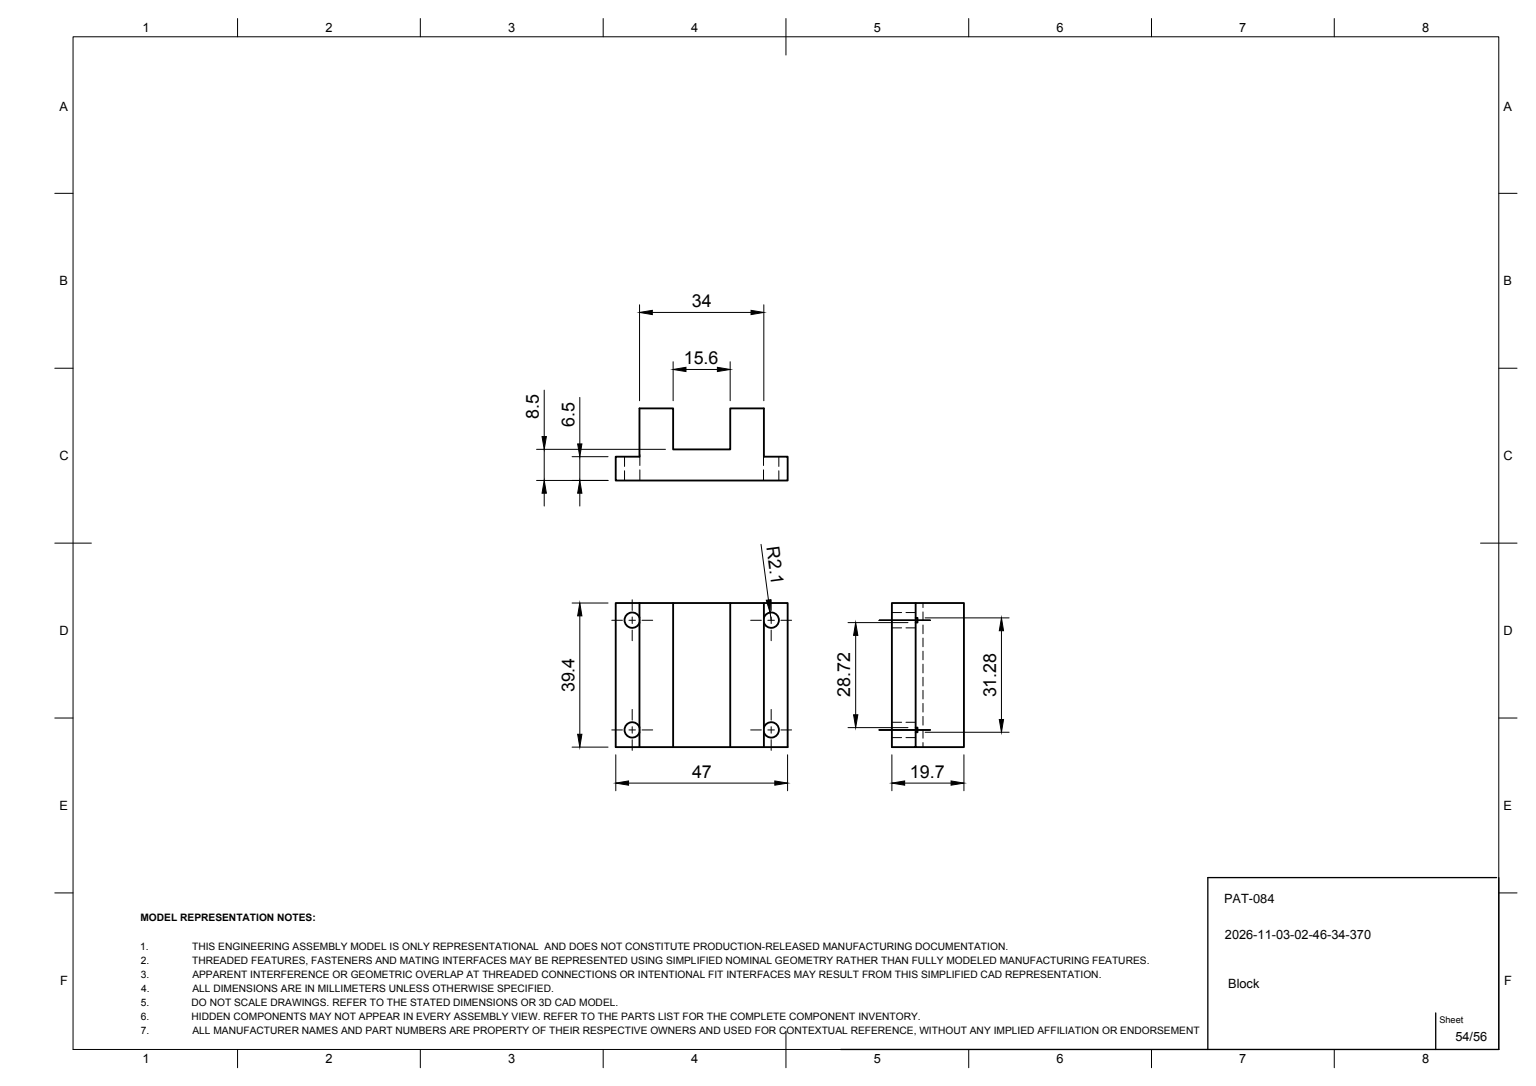
ISO-10303-21;
HEADER;
/* Generated by software containing ST-Developer
 * from STEP Tools, Inc. (www.steptools.com) 
 */

FILE_DESCRIPTION(
/* description */ ('Quick-return (Whitworth) mechanism'),
/* implementation_level */ '2;1');

FILE_NAME(
/* name */ 'Block.step',
/* time_stamp */ '2026-10-28T03:25:57-07:00',
/* author */ (''),
/* organization */ (''),
/* preprocessor_version */ 'ST-DEVELOPER v20.2',
/* originating_system */ 'Autodesk Translation Framework v15.17.0.0',
/* authorisation */ '');

FILE_SCHEMA (('AUTOMOTIVE_DESIGN { 1 0 10303 214 3 1 1 }'));
ENDSEC;

DATA;
#10=MECHANICAL_DESIGN_GEOMETRIC_PRESENTATION_REPRESENTATION('',(#537),#14878);
#441=SHAPE_REPRESENTATION_RELATIONSHIP('SRR','None',#15116,#485);
#485=ADVANCED_BREP_SHAPE_REPRESENTATION('',(#588),#14873);
#537=STYLED_ITEM('',(#15385),#588);
#588=MANIFOLD_SOLID_BREP('Body1',#7892);
#776=FACE_BOUND('',#2104,.T.);
#777=FACE_BOUND('',#2105,.T.);
#778=FACE_BOUND('',#2106,.T.);
#779=FACE_BOUND('',#2107,.T.);
#987=PLANE('',#9219);
#988=PLANE('',#9225);
#989=PLANE('',#9231);
#990=PLANE('',#9237);
#991=PLANE('',#9243);
#992=PLANE('',#9244);
#993=PLANE('',#9245);
#994=PLANE('',#9246);
#995=PLANE('',#9247);
#996=PLANE('',#9248);
#997=PLANE('',#9249);
#998=PLANE('',#9250);
#999=PLANE('',#9251);
#1000=PLANE('',#9252);
#1001=PLANE('',#9253);
#1002=PLANE('',#9254);
#1003=PLANE('',#9255);
#1004=PLANE('',#9256);
#1439=FACE_OUTER_BOUND('',#2090,.T.);
#1440=FACE_OUTER_BOUND('',#2091,.T.);
#1441=FACE_OUTER_BOUND('',#2092,.T.);
#1442=FACE_OUTER_BOUND('',#2093,.T.);
#1443=FACE_OUTER_BOUND('',#2094,.T.);
#1444=FACE_OUTER_BOUND('',#2095,.T.);
#1445=FACE_OUTER_BOUND('',#2096,.T.);
#1446=FACE_OUTER_BOUND('',#2097,.T.);
#1447=FACE_OUTER_BOUND('',#2098,.T.);
#1448=FACE_OUTER_BOUND('',#2099,.T.);
#1449=FACE_OUTER_BOUND('',#2100,.T.);
#1450=FACE_OUTER_BOUND('',#2101,.T.);
#1451=FACE_OUTER_BOUND('',#2102,.T.);
#1452=FACE_OUTER_BOUND('',#2103,.T.);
#1453=FACE_OUTER_BOUND('',#2108,.T.);
#1454=FACE_OUTER_BOUND('',#2109,.T.);
#1455=FACE_OUTER_BOUND('',#2110,.T.);
#1456=FACE_OUTER_BOUND('',#2111,.T.);
#1457=FACE_OUTER_BOUND('',#2112,.T.);
#1458=FACE_OUTER_BOUND('',#2113,.T.);
#1459=FACE_OUTER_BOUND('',#2114,.T.);
#1460=FACE_OUTER_BOUND('',#2115,.T.);
#2090=EDGE_LOOP('',(#6850,#6851));
#2091=EDGE_LOOP('',(#6852,#6853,#6854,#6855,#6856,#6857,#6858,#6859));
#2092=EDGE_LOOP('',(#6860,#6861));
#2093=EDGE_LOOP('',(#6862,#6863,#6864,#6865,#6866,#6867,#6868,#6869));
#2094=EDGE_LOOP('',(#6870,#6871));
#2095=EDGE_LOOP('',(#6872,#6873,#6874,#6875,#6876,#6877,#6878,#6879));
#2096=EDGE_LOOP('',(#6880,#6881));
#2097=EDGE_LOOP('',(#6882,#6883,#6884,#6885,#6886,#6887,#6888,#6889));
#2098=EDGE_LOOP('',(#6890,#6891,#6892,#6893,#6894,#6895,#6896,#6897,#6898,
#6899,#6900,#6901));
#2099=EDGE_LOOP('',(#6902,#6903,#6904,#6905,#6906,#6907,#6908,#6909,#6910,
#6911,#6912,#6913));
#2100=EDGE_LOOP('',(#6914,#6915,#6916,#6917,#6918,#6919,#6920,#6921,#6922,
#6923,#6924,#6925));
#2101=EDGE_LOOP('',(#6926,#6927,#6928,#6929,#6930,#6931,#6932,#6933,#6934,
#6935));
#2102=EDGE_LOOP('',(#6936,#6937,#6938,#6939));
#2103=EDGE_LOOP('',(#6940,#6941,#6942,#6943));
#2104=EDGE_LOOP('',(#6944));
#2105=EDGE_LOOP('',(#6945));
#2106=EDGE_LOOP('',(#6946));
#2107=EDGE_LOOP('',(#6947));
#2108=EDGE_LOOP('',(#6948,#6949,#6950,#6951));
#2109=EDGE_LOOP('',(#6952,#6953,#6954,#6955,#6956,#6957,#6958,#6959,#6960,
#6961));
#2110=EDGE_LOOP('',(#6962,#6963,#6964,#6965));
#2111=EDGE_LOOP('',(#6966,#6967,#6968,#6969));
#2112=EDGE_LOOP('',(#6970,#6971,#6972,#6973));
#2113=EDGE_LOOP('',(#6974,#6975,#6976,#6977));
#2114=EDGE_LOOP('',(#6978,#6979,#6980,#6981));
#2115=EDGE_LOOP('',(#6982,#6983,#6984,#6985,#6986,#6987,#6988,#6989,#6990,
#6991,#6992,#6993));
#2543=LINE('',#14328,#3066);
#2544=LINE('',#14332,#3067);
#2545=LINE('',#14336,#3068);
#2546=LINE('',#14340,#3069);
#2547=LINE('',#14344,#3070);
#2548=LINE('',#14348,#3071);
#2549=LINE('',#14352,#3072);
#2550=LINE('',#14356,#3073);
#2551=LINE('',#14360,#3074);
#2552=LINE('',#14364,#3075);
#2553=LINE('',#14368,#3076);
#2554=LINE('',#14372,#3077);
#2555=LINE('',#14376,#3078);
#2556=LINE('',#14380,#3079);
#2557=LINE('',#14384,#3080);
#2558=LINE('',#14388,#3081);
#2559=LINE('',#14390,#3082);
#2560=LINE('',#14392,#3083);
#2561=LINE('',#14394,#3084);
#2562=LINE('',#14396,#3085);
#2563=LINE('',#14398,#3086);
#2564=LINE('',#14399,#3087);
#2565=LINE('',#14401,#3088);
#2566=LINE('',#14403,#3089);
#2567=LINE('',#14405,#3090);
#2568=LINE('',#14407,#3091);
#2569=LINE('',#14409,#3092);
#2570=LINE('',#14410,#3093);
#2571=LINE('',#14413,#3094);
#2572=LINE('',#14415,#3095);
#2573=LINE('',#14417,#3096);
#2574=LINE('',#14419,#3097);
#2575=LINE('',#14420,#3098);
#2576=LINE('',#14422,#3099);
#2577=LINE('',#14424,#3100);
#2578=LINE('',#14426,#3101);
#2579=LINE('',#14428,#3102);
#2580=LINE('',#14429,#3103);
#2581=LINE('',#14432,#3104);
#2582=LINE('',#14433,#3105);
#2583=LINE('',#14436,#3106);
#2584=LINE('',#14437,#3107);
#2585=LINE('',#14440,#3108);
#2586=LINE('',#14441,#3109);
#2587=LINE('',#14444,#3110);
#2588=LINE('',#14445,#3111);
#2589=LINE('',#14447,#3112);
#2590=LINE('',#14450,#3113);
#2591=LINE('',#14451,#3114);
#2592=LINE('',#14454,#3115);
#2593=LINE('',#14455,#3116);
#2594=LINE('',#14458,#3117);
#2595=LINE('',#14459,#3118);
#2596=LINE('',#14462,#3119);
#2597=LINE('',#14463,#3120);
#2598=LINE('',#14465,#3121);
#3066=VECTOR('',#11442,1.);
#3067=VECTOR('',#11447,1.);
#3068=VECTOR('',#11450,0.21);
#3069=VECTOR('',#11455,1.);
#3070=VECTOR('',#11458,1.);
#3071=VECTOR('',#11463,1.);
#3072=VECTOR('',#11466,0.21);
#3073=VECTOR('',#11471,1.);
#3074=VECTOR('',#11474,1.);
#3075=VECTOR('',#11479,1.);
#3076=VECTOR('',#11482,0.21);
#3077=VECTOR('',#11487,1.);
#3078=VECTOR('',#11490,1.);
#3079=VECTOR('',#11495,1.);
#3080=VECTOR('',#11498,0.21);
#3081=VECTOR('',#11503,1.);
#3082=VECTOR('',#11506,1.);
#3083=VECTOR('',#11507,1.);
#3084=VECTOR('',#11508,1.);
#3085=VECTOR('',#11509,1.);
#3086=VECTOR('',#11510,1.);
#3087=VECTOR('',#11511,1.);
#3088=VECTOR('',#11514,1.);
#3089=VECTOR('',#11515,1.);
#3090=VECTOR('',#11516,1.);
#3091=VECTOR('',#11517,1.);
#3092=VECTOR('',#11518,1.);
#3093=VECTOR('',#11519,1.);
#3094=VECTOR('',#11522,1.);
#3095=VECTOR('',#11523,1.);
#3096=VECTOR('',#11524,1.);
#3097=VECTOR('',#11525,1.);
#3098=VECTOR('',#11526,1.);
#3099=VECTOR('',#11527,1.);
#3100=VECTOR('',#11528,1.);
#3101=VECTOR('',#11529,1.);
#3102=VECTOR('',#11530,1.);
#3103=VECTOR('',#11531,1.);
#3104=VECTOR('',#11534,1.);
#3105=VECTOR('',#11535,1.);
#3106=VECTOR('',#11538,1.);
#3107=VECTOR('',#11539,1.);
#3108=VECTOR('',#11542,1.);
#3109=VECTOR('',#11543,1.);
#3110=VECTOR('',#11546,1.);
#3111=VECTOR('',#11547,1.);
#3112=VECTOR('',#11550,1.);
#3113=VECTOR('',#11553,1.);
#3114=VECTOR('',#11554,1.);
#3115=VECTOR('',#11557,1.);
#3116=VECTOR('',#11558,1.);
#3117=VECTOR('',#11561,1.);
#3118=VECTOR('',#11562,1.);
#3119=VECTOR('',#11565,1.);
#3120=VECTOR('',#11566,1.);
#3121=VECTOR('',#11569,1.);
#3601=CIRCLE('',#9220,0.21);
#3602=CIRCLE('',#9222,0.21);
#3603=CIRCLE('',#9223,0.21);
#3604=CIRCLE('',#9224,0.21);
#3605=CIRCLE('',#9226,0.21);
#3606=CIRCLE('',#9228,0.21);
#3607=CIRCLE('',#9229,0.21);
#3608=CIRCLE('',#9230,0.21);
#3609=CIRCLE('',#9232,0.21);
#3610=CIRCLE('',#9234,0.21);
#3611=CIRCLE('',#9235,0.21);
#3612=CIRCLE('',#9236,0.21);
#3613=CIRCLE('',#9238,0.21);
#3614=CIRCLE('',#9240,0.21);
#3615=CIRCLE('',#9241,0.21);
#3616=CIRCLE('',#9242,0.21);
#4170=VERTEX_POINT('',#14326);
#4171=VERTEX_POINT('',#14327);
#4172=VERTEX_POINT('',#14331);
#4173=VERTEX_POINT('',#14333);
#4174=VERTEX_POINT('',#14335);
#4175=VERTEX_POINT('',#14338);
#4176=VERTEX_POINT('',#14342);
#4177=VERTEX_POINT('',#14343);
#4178=VERTEX_POINT('',#14347);
#4179=VERTEX_POINT('',#14349);
#4180=VERTEX_POINT('',#14351);
#4181=VERTEX_POINT('',#14354);
#4182=VERTEX_POINT('',#14358);
#4183=VERTEX_POINT('',#14359);
#4184=VERTEX_POINT('',#14363);
#4185=VERTEX_POINT('',#14365);
#4186=VERTEX_POINT('',#14367);
#4187=VERTEX_POINT('',#14370);
#4188=VERTEX_POINT('',#14374);
#4189=VERTEX_POINT('',#14375);
#4190=VERTEX_POINT('',#14379);
#4191=VERTEX_POINT('',#14381);
#4192=VERTEX_POINT('',#14383);
#4193=VERTEX_POINT('',#14386);
#4194=VERTEX_POINT('',#14391);
#4195=VERTEX_POINT('',#14393);
#4196=VERTEX_POINT('',#14395);
#4197=VERTEX_POINT('',#14397);
#4198=VERTEX_POINT('',#14402);
#4199=VERTEX_POINT('',#14404);
#4200=VERTEX_POINT('',#14406);
#4201=VERTEX_POINT('',#14408);
#4202=VERTEX_POINT('',#14412);
#4203=VERTEX_POINT('',#14414);
#4204=VERTEX_POINT('',#14416);
#4205=VERTEX_POINT('',#14418);
#4206=VERTEX_POINT('',#14421);
#4207=VERTEX_POINT('',#14423);
#4208=VERTEX_POINT('',#14425);
#4209=VERTEX_POINT('',#14427);
#4210=VERTEX_POINT('',#14431);
#4211=VERTEX_POINT('',#14435);
#4212=VERTEX_POINT('',#14439);
#4213=VERTEX_POINT('',#14443);
#4214=VERTEX_POINT('',#14449);
#4215=VERTEX_POINT('',#14453);
#4216=VERTEX_POINT('',#14457);
#4217=VERTEX_POINT('',#14461);
#5082=EDGE_CURVE('',#4170,#4171,#2543,.T.);
#5083=EDGE_CURVE('',#4170,#4171,#3601,.T.);
#5084=EDGE_CURVE('',#4172,#4170,#2544,.T.);
#5085=EDGE_CURVE('',#4173,#4172,#3602,.T.);
#5086=EDGE_CURVE('',#4173,#4174,#2545,.T.);
#5087=EDGE_CURVE('',#4174,#4174,#3603,.T.);
#5088=EDGE_CURVE('',#4175,#4173,#3604,.T.);
#5089=EDGE_CURVE('',#4171,#4175,#2546,.T.);
#5090=EDGE_CURVE('',#4176,#4177,#2547,.T.);
#5091=EDGE_CURVE('',#4176,#4177,#3605,.T.);
#5092=EDGE_CURVE('',#4178,#4176,#2548,.T.);
#5093=EDGE_CURVE('',#4179,#4178,#3606,.T.);
#5094=EDGE_CURVE('',#4179,#4180,#2549,.T.);
#5095=EDGE_CURVE('',#4180,#4180,#3607,.T.);
#5096=EDGE_CURVE('',#4181,#4179,#3608,.T.);
#5097=EDGE_CURVE('',#4177,#4181,#2550,.T.);
#5098=EDGE_CURVE('',#4182,#4183,#2551,.T.);
#5099=EDGE_CURVE('',#4182,#4183,#3609,.T.);
#5100=EDGE_CURVE('',#4184,#4182,#2552,.T.);
#5101=EDGE_CURVE('',#4185,#4184,#3610,.T.);
#5102=EDGE_CURVE('',#4185,#4186,#2553,.T.);
#5103=EDGE_CURVE('',#4186,#4186,#3611,.T.);
#5104=EDGE_CURVE('',#4187,#4185,#3612,.T.);
#5105=EDGE_CURVE('',#4183,#4187,#2554,.T.);
#5106=EDGE_CURVE('',#4188,#4189,#2555,.T.);
#5107=EDGE_CURVE('',#4188,#4189,#3613,.T.);
#5108=EDGE_CURVE('',#4190,#4188,#2556,.T.);
#5109=EDGE_CURVE('',#4191,#4190,#3614,.T.);
#5110=EDGE_CURVE('',#4191,#4192,#2557,.T.);
#5111=EDGE_CURVE('',#4192,#4192,#3615,.T.);
#5112=EDGE_CURVE('',#4193,#4191,#3616,.T.);
#5113=EDGE_CURVE('',#4189,#4193,#2558,.T.);
#5114=EDGE_CURVE('',#4175,#4184,#2559,.T.);
#5115=EDGE_CURVE('',#4187,#4194,#2560,.T.);
#5116=EDGE_CURVE('',#4195,#4194,#2561,.T.);
#5117=EDGE_CURVE('',#4195,#4196,#2562,.T.);
#5118=EDGE_CURVE('',#4197,#4196,#2563,.T.);
#5119=EDGE_CURVE('',#4197,#4172,#2564,.T.);
#5120=EDGE_CURVE('',#4181,#4190,#2565,.T.);
#5121=EDGE_CURVE('',#4193,#4198,#2566,.T.);
#5122=EDGE_CURVE('',#4199,#4198,#2567,.T.);
#5123=EDGE_CURVE('',#4200,#4199,#2568,.T.);
#5124=EDGE_CURVE('',#4201,#4200,#2569,.T.);
#5125=EDGE_CURVE('',#4201,#4178,#2570,.T.);
#5126=EDGE_CURVE('',#4194,#4202,#2571,.T.);
#5127=EDGE_CURVE('',#4202,#4203,#2572,.T.);
#5128=EDGE_CURVE('',#4203,#4204,#2573,.T.);
#5129=EDGE_CURVE('',#4204,#4205,#2574,.T.);
#5130=EDGE_CURVE('',#4205,#4201,#2575,.T.);
#5131=EDGE_CURVE('',#4200,#4206,#2576,.T.);
#5132=EDGE_CURVE('',#4206,#4207,#2577,.T.);
#5133=EDGE_CURVE('',#4207,#4208,#2578,.T.);
#5134=EDGE_CURVE('',#4208,#4209,#2579,.T.);
#5135=EDGE_CURVE('',#4209,#4195,#2580,.T.);
#5136=EDGE_CURVE('',#4210,#4197,#2581,.T.);
#5137=EDGE_CURVE('',#4202,#4210,#2582,.T.);
#5138=EDGE_CURVE('',#4211,#4210,#2583,.T.);
#5139=EDGE_CURVE('',#4203,#4211,#2584,.T.);
#5140=EDGE_CURVE('',#4212,#4211,#2585,.T.);
#5141=EDGE_CURVE('',#4204,#4212,#2586,.T.);
#5142=EDGE_CURVE('',#4213,#4212,#2587,.T.);
#5143=EDGE_CURVE('',#4205,#4213,#2588,.T.);
#5144=EDGE_CURVE('',#4198,#4213,#2589,.T.);
#5145=EDGE_CURVE('',#4214,#4199,#2590,.T.);
#5146=EDGE_CURVE('',#4206,#4214,#2591,.T.);
#5147=EDGE_CURVE('',#4215,#4214,#2592,.T.);
#5148=EDGE_CURVE('',#4207,#4215,#2593,.T.);
#5149=EDGE_CURVE('',#4216,#4215,#2594,.T.);
#5150=EDGE_CURVE('',#4208,#4216,#2595,.T.);
#5151=EDGE_CURVE('',#4217,#4216,#2596,.T.);
#5152=EDGE_CURVE('',#4209,#4217,#2597,.T.);
#5153=EDGE_CURVE('',#4196,#4217,#2598,.T.);
#6850=ORIENTED_EDGE('',*,*,#5082,.F.);
#6851=ORIENTED_EDGE('',*,*,#5083,.T.);
#6852=ORIENTED_EDGE('',*,*,#5084,.F.);
#6853=ORIENTED_EDGE('',*,*,#5085,.F.);
#6854=ORIENTED_EDGE('',*,*,#5086,.T.);
#6855=ORIENTED_EDGE('',*,*,#5087,.F.);
#6856=ORIENTED_EDGE('',*,*,#5086,.F.);
#6857=ORIENTED_EDGE('',*,*,#5088,.F.);
#6858=ORIENTED_EDGE('',*,*,#5089,.F.);
#6859=ORIENTED_EDGE('',*,*,#5083,.F.);
#6860=ORIENTED_EDGE('',*,*,#5090,.F.);
#6861=ORIENTED_EDGE('',*,*,#5091,.T.);
#6862=ORIENTED_EDGE('',*,*,#5092,.F.);
#6863=ORIENTED_EDGE('',*,*,#5093,.F.);
#6864=ORIENTED_EDGE('',*,*,#5094,.T.);
#6865=ORIENTED_EDGE('',*,*,#5095,.F.);
#6866=ORIENTED_EDGE('',*,*,#5094,.F.);
#6867=ORIENTED_EDGE('',*,*,#5096,.F.);
#6868=ORIENTED_EDGE('',*,*,#5097,.F.);
#6869=ORIENTED_EDGE('',*,*,#5091,.F.);
#6870=ORIENTED_EDGE('',*,*,#5098,.F.);
#6871=ORIENTED_EDGE('',*,*,#5099,.T.);
#6872=ORIENTED_EDGE('',*,*,#5100,.F.);
#6873=ORIENTED_EDGE('',*,*,#5101,.F.);
#6874=ORIENTED_EDGE('',*,*,#5102,.T.);
#6875=ORIENTED_EDGE('',*,*,#5103,.F.);
#6876=ORIENTED_EDGE('',*,*,#5102,.F.);
#6877=ORIENTED_EDGE('',*,*,#5104,.F.);
#6878=ORIENTED_EDGE('',*,*,#5105,.F.);
#6879=ORIENTED_EDGE('',*,*,#5099,.F.);
#6880=ORIENTED_EDGE('',*,*,#5106,.F.);
#6881=ORIENTED_EDGE('',*,*,#5107,.T.);
#6882=ORIENTED_EDGE('',*,*,#5108,.F.);
#6883=ORIENTED_EDGE('',*,*,#5109,.F.);
#6884=ORIENTED_EDGE('',*,*,#5110,.T.);
#6885=ORIENTED_EDGE('',*,*,#5111,.F.);
#6886=ORIENTED_EDGE('',*,*,#5110,.F.);
#6887=ORIENTED_EDGE('',*,*,#5112,.F.);
#6888=ORIENTED_EDGE('',*,*,#5113,.F.);
#6889=ORIENTED_EDGE('',*,*,#5107,.F.);
#6890=ORIENTED_EDGE('',*,*,#5084,.T.);
#6891=ORIENTED_EDGE('',*,*,#5082,.T.);
#6892=ORIENTED_EDGE('',*,*,#5089,.T.);
#6893=ORIENTED_EDGE('',*,*,#5114,.T.);
#6894=ORIENTED_EDGE('',*,*,#5100,.T.);
#6895=ORIENTED_EDGE('',*,*,#5098,.T.);
#6896=ORIENTED_EDGE('',*,*,#5105,.T.);
#6897=ORIENTED_EDGE('',*,*,#5115,.T.);
#6898=ORIENTED_EDGE('',*,*,#5116,.F.);
#6899=ORIENTED_EDGE('',*,*,#5117,.T.);
#6900=ORIENTED_EDGE('',*,*,#5118,.F.);
#6901=ORIENTED_EDGE('',*,*,#5119,.T.);
#6902=ORIENTED_EDGE('',*,*,#5092,.T.);
#6903=ORIENTED_EDGE('',*,*,#5090,.T.);
#6904=ORIENTED_EDGE('',*,*,#5097,.T.);
#6905=ORIENTED_EDGE('',*,*,#5120,.T.);
#6906=ORIENTED_EDGE('',*,*,#5108,.T.);
#6907=ORIENTED_EDGE('',*,*,#5106,.T.);
#6908=ORIENTED_EDGE('',*,*,#5113,.T.);
#6909=ORIENTED_EDGE('',*,*,#5121,.T.);
#6910=ORIENTED_EDGE('',*,*,#5122,.F.);
#6911=ORIENTED_EDGE('',*,*,#5123,.F.);
#6912=ORIENTED_EDGE('',*,*,#5124,.F.);
#6913=ORIENTED_EDGE('',*,*,#5125,.T.);
#6914=ORIENTED_EDGE('',*,*,#5116,.T.);
#6915=ORIENTED_EDGE('',*,*,#5126,.T.);
#6916=ORIENTED_EDGE('',*,*,#5127,.T.);
#6917=ORIENTED_EDGE('',*,*,#5128,.T.);
#6918=ORIENTED_EDGE('',*,*,#5129,.T.);
#6919=ORIENTED_EDGE('',*,*,#5130,.T.);
#6920=ORIENTED_EDGE('',*,*,#5124,.T.);
#6921=ORIENTED_EDGE('',*,*,#5131,.T.);
#6922=ORIENTED_EDGE('',*,*,#5132,.T.);
#6923=ORIENTED_EDGE('',*,*,#5133,.T.);
#6924=ORIENTED_EDGE('',*,*,#5134,.T.);
#6925=ORIENTED_EDGE('',*,*,#5135,.T.);
#6926=ORIENTED_EDGE('',*,*,#5088,.T.);
#6927=ORIENTED_EDGE('',*,*,#5085,.T.);
#6928=ORIENTED_EDGE('',*,*,#5119,.F.);
#6929=ORIENTED_EDGE('',*,*,#5136,.F.);
#6930=ORIENTED_EDGE('',*,*,#5137,.F.);
#6931=ORIENTED_EDGE('',*,*,#5126,.F.);
#6932=ORIENTED_EDGE('',*,*,#5115,.F.);
#6933=ORIENTED_EDGE('',*,*,#5104,.T.);
#6934=ORIENTED_EDGE('',*,*,#5101,.T.);
#6935=ORIENTED_EDGE('',*,*,#5114,.F.);
#6936=ORIENTED_EDGE('',*,*,#5137,.T.);
#6937=ORIENTED_EDGE('',*,*,#5138,.F.);
#6938=ORIENTED_EDGE('',*,*,#5139,.F.);
#6939=ORIENTED_EDGE('',*,*,#5127,.F.);
#6940=ORIENTED_EDGE('',*,*,#5139,.T.);
#6941=ORIENTED_EDGE('',*,*,#5140,.F.);
#6942=ORIENTED_EDGE('',*,*,#5141,.F.);
#6943=ORIENTED_EDGE('',*,*,#5128,.F.);
#6944=ORIENTED_EDGE('',*,*,#5087,.T.);
#6945=ORIENTED_EDGE('',*,*,#5095,.T.);
#6946=ORIENTED_EDGE('',*,*,#5103,.T.);
#6947=ORIENTED_EDGE('',*,*,#5111,.T.);
#6948=ORIENTED_EDGE('',*,*,#5141,.T.);
#6949=ORIENTED_EDGE('',*,*,#5142,.F.);
#6950=ORIENTED_EDGE('',*,*,#5143,.F.);
#6951=ORIENTED_EDGE('',*,*,#5129,.F.);
#6952=ORIENTED_EDGE('',*,*,#5096,.T.);
#6953=ORIENTED_EDGE('',*,*,#5093,.T.);
#6954=ORIENTED_EDGE('',*,*,#5125,.F.);
#6955=ORIENTED_EDGE('',*,*,#5130,.F.);
#6956=ORIENTED_EDGE('',*,*,#5143,.T.);
#6957=ORIENTED_EDGE('',*,*,#5144,.F.);
#6958=ORIENTED_EDGE('',*,*,#5121,.F.);
#6959=ORIENTED_EDGE('',*,*,#5112,.T.);
#6960=ORIENTED_EDGE('',*,*,#5109,.T.);
#6961=ORIENTED_EDGE('',*,*,#5120,.F.);
#6962=ORIENTED_EDGE('',*,*,#5123,.T.);
#6963=ORIENTED_EDGE('',*,*,#5145,.F.);
#6964=ORIENTED_EDGE('',*,*,#5146,.F.);
#6965=ORIENTED_EDGE('',*,*,#5131,.F.);
#6966=ORIENTED_EDGE('',*,*,#5146,.T.);
#6967=ORIENTED_EDGE('',*,*,#5147,.F.);
#6968=ORIENTED_EDGE('',*,*,#5148,.F.);
#6969=ORIENTED_EDGE('',*,*,#5132,.F.);
#6970=ORIENTED_EDGE('',*,*,#5148,.T.);
#6971=ORIENTED_EDGE('',*,*,#5149,.F.);
#6972=ORIENTED_EDGE('',*,*,#5150,.F.);
#6973=ORIENTED_EDGE('',*,*,#5133,.F.);
#6974=ORIENTED_EDGE('',*,*,#5150,.T.);
#6975=ORIENTED_EDGE('',*,*,#5151,.F.);
#6976=ORIENTED_EDGE('',*,*,#5152,.F.);
#6977=ORIENTED_EDGE('',*,*,#5134,.F.);
#6978=ORIENTED_EDGE('',*,*,#5152,.T.);
#6979=ORIENTED_EDGE('',*,*,#5153,.F.);
#6980=ORIENTED_EDGE('',*,*,#5117,.F.);
#6981=ORIENTED_EDGE('',*,*,#5135,.F.);
#6982=ORIENTED_EDGE('',*,*,#5118,.T.);
#6983=ORIENTED_EDGE('',*,*,#5153,.T.);
#6984=ORIENTED_EDGE('',*,*,#5151,.T.);
#6985=ORIENTED_EDGE('',*,*,#5149,.T.);
#6986=ORIENTED_EDGE('',*,*,#5147,.T.);
#6987=ORIENTED_EDGE('',*,*,#5145,.T.);
#6988=ORIENTED_EDGE('',*,*,#5122,.T.);
#6989=ORIENTED_EDGE('',*,*,#5144,.T.);
#6990=ORIENTED_EDGE('',*,*,#5142,.T.);
#6991=ORIENTED_EDGE('',*,*,#5140,.T.);
#6992=ORIENTED_EDGE('',*,*,#5138,.T.);
#6993=ORIENTED_EDGE('',*,*,#5136,.T.);
#7370=CYLINDRICAL_SURFACE('',#9221,0.21);
#7371=CYLINDRICAL_SURFACE('',#9227,0.21);
#7372=CYLINDRICAL_SURFACE('',#9233,0.21);
#7373=CYLINDRICAL_SURFACE('',#9239,0.21);
#7770=ADVANCED_FACE('',(#1439),#987,.T.);
#7771=ADVANCED_FACE('',(#1440),#7370,.F.);
#7772=ADVANCED_FACE('',(#1441),#988,.T.);
#7773=ADVANCED_FACE('',(#1442),#7371,.F.);
#7774=ADVANCED_FACE('',(#1443),#989,.T.);
#7775=ADVANCED_FACE('',(#1444),#7372,.F.);
#7776=ADVANCED_FACE('',(#1445),#990,.T.);
#7777=ADVANCED_FACE('',(#1446),#7373,.F.);
#7778=ADVANCED_FACE('',(#1447),#991,.T.);
#7779=ADVANCED_FACE('',(#1448),#992,.T.);
#7780=ADVANCED_FACE('',(#1449),#993,.T.);
#7781=ADVANCED_FACE('',(#1450),#994,.T.);
#7782=ADVANCED_FACE('',(#1451),#995,.T.);
#7783=ADVANCED_FACE('',(#1452,#776,#777,#778,#779),#996,.T.);
#7784=ADVANCED_FACE('',(#1453),#997,.T.);
#7785=ADVANCED_FACE('',(#1454),#998,.T.);
#7786=ADVANCED_FACE('',(#1455),#999,.T.);
#7787=ADVANCED_FACE('',(#1456),#1000,.T.);
#7788=ADVANCED_FACE('',(#1457),#1001,.T.);
#7789=ADVANCED_FACE('',(#1458),#1002,.T.);
#7790=ADVANCED_FACE('',(#1459),#1003,.T.);
#7791=ADVANCED_FACE('',(#1460),#1004,.T.);
#7892=CLOSED_SHELL('',(#7770,#7771,#7772,#7773,#7774,#7775,#7776,#7777,
#7778,#7779,#7780,#7781,#7782,#7783,#7784,#7785,#7786,#7787,#7788,#7789,
#7790,#7791));
#9218=AXIS2_PLACEMENT_3D('',#14324,#11438,#11439);
#9219=AXIS2_PLACEMENT_3D('',#14325,#11440,#11441);
#9220=AXIS2_PLACEMENT_3D('',#14329,#11443,#11444);
#9221=AXIS2_PLACEMENT_3D('',#14330,#11445,#11446);
#9222=AXIS2_PLACEMENT_3D('',#14334,#11448,#11449);
#9223=AXIS2_PLACEMENT_3D('',#14337,#11451,#11452);
#9224=AXIS2_PLACEMENT_3D('',#14339,#11453,#11454);
#9225=AXIS2_PLACEMENT_3D('',#14341,#11456,#11457);
#9226=AXIS2_PLACEMENT_3D('',#14345,#11459,#11460);
#9227=AXIS2_PLACEMENT_3D('',#14346,#11461,#11462);
#9228=AXIS2_PLACEMENT_3D('',#14350,#11464,#11465);
#9229=AXIS2_PLACEMENT_3D('',#14353,#11467,#11468);
#9230=AXIS2_PLACEMENT_3D('',#14355,#11469,#11470);
#9231=AXIS2_PLACEMENT_3D('',#14357,#11472,#11473);
#9232=AXIS2_PLACEMENT_3D('',#14361,#11475,#11476);
#9233=AXIS2_PLACEMENT_3D('',#14362,#11477,#11478);
#9234=AXIS2_PLACEMENT_3D('',#14366,#11480,#11481);
#9235=AXIS2_PLACEMENT_3D('',#14369,#11483,#11484);
#9236=AXIS2_PLACEMENT_3D('',#14371,#11485,#11486);
#9237=AXIS2_PLACEMENT_3D('',#14373,#11488,#11489);
#9238=AXIS2_PLACEMENT_3D('',#14377,#11491,#11492);
#9239=AXIS2_PLACEMENT_3D('',#14378,#11493,#11494);
#9240=AXIS2_PLACEMENT_3D('',#14382,#11496,#11497);
#9241=AXIS2_PLACEMENT_3D('',#14385,#11499,#11500);
#9242=AXIS2_PLACEMENT_3D('',#14387,#11501,#11502);
#9243=AXIS2_PLACEMENT_3D('',#14389,#11504,#11505);
#9244=AXIS2_PLACEMENT_3D('',#14400,#11512,#11513);
#9245=AXIS2_PLACEMENT_3D('',#14411,#11520,#11521);
#9246=AXIS2_PLACEMENT_3D('',#14430,#11532,#11533);
#9247=AXIS2_PLACEMENT_3D('',#14434,#11536,#11537);
#9248=AXIS2_PLACEMENT_3D('',#14438,#11540,#11541);
#9249=AXIS2_PLACEMENT_3D('',#14442,#11544,#11545);
#9250=AXIS2_PLACEMENT_3D('',#14446,#11548,#11549);
#9251=AXIS2_PLACEMENT_3D('',#14448,#11551,#11552);
#9252=AXIS2_PLACEMENT_3D('',#14452,#11555,#11556);
#9253=AXIS2_PLACEMENT_3D('',#14456,#11559,#11560);
#9254=AXIS2_PLACEMENT_3D('',#14460,#11563,#11564);
#9255=AXIS2_PLACEMENT_3D('',#14464,#11567,#11568);
#9256=AXIS2_PLACEMENT_3D('',#14466,#11570,#11571);
#11438=DIRECTION('axis',(0.,0.,1.));
#11439=DIRECTION('refdir',(1.,0.,0.));
#11440=DIRECTION('center_axis',(0.,0.,1.));
#11441=DIRECTION('ref_axis',(1.,0.,0.));
#11442=DIRECTION('',(-1.,0.,0.));
#11443=DIRECTION('center_axis',(0.,0.,1.));
#11444=DIRECTION('ref_axis',(1.,0.,0.));
#11445=DIRECTION('center_axis',(0.,0.,1.));
#11446=DIRECTION('ref_axis',(1.,0.,0.));
#11447=DIRECTION('',(0.,0.,-1.));
#11448=DIRECTION('center_axis',(0.,0.,1.));
#11449=DIRECTION('ref_axis',(1.,0.,0.));
#11450=DIRECTION('',(0.,0.,1.));
#11451=DIRECTION('center_axis',(0.,0.,-1.));
#11452=DIRECTION('ref_axis',(1.,0.,0.));
#11453=DIRECTION('center_axis',(0.,0.,1.));
#11454=DIRECTION('ref_axis',(1.,0.,0.));
#11455=DIRECTION('',(0.,0.,1.));
#11456=DIRECTION('center_axis',(0.,0.,1.));
#11457=DIRECTION('ref_axis',(1.,0.,0.));
#11458=DIRECTION('',(1.,0.,0.));
#11459=DIRECTION('center_axis',(0.,0.,1.));
#11460=DIRECTION('ref_axis',(1.,0.,0.));
#11461=DIRECTION('center_axis',(0.,0.,1.));
#11462=DIRECTION('ref_axis',(1.,0.,0.));
#11463=DIRECTION('',(0.,0.,-1.));
#11464=DIRECTION('center_axis',(0.,0.,1.));
#11465=DIRECTION('ref_axis',(1.,0.,0.));
#11466=DIRECTION('',(0.,0.,1.));
#11467=DIRECTION('center_axis',(0.,0.,-1.));
#11468=DIRECTION('ref_axis',(1.,0.,0.));
#11469=DIRECTION('center_axis',(0.,0.,1.));
#11470=DIRECTION('ref_axis',(1.,0.,0.));
#11471=DIRECTION('',(0.,0.,1.));
#11472=DIRECTION('center_axis',(0.,0.,1.));
#11473=DIRECTION('ref_axis',(1.,0.,0.));
#11474=DIRECTION('',(-1.,0.,0.));
#11475=DIRECTION('center_axis',(0.,0.,1.));
#11476=DIRECTION('ref_axis',(1.,0.,0.));
#11477=DIRECTION('center_axis',(0.,0.,1.));
#11478=DIRECTION('ref_axis',(1.,0.,0.));
#11479=DIRECTION('',(0.,0.,-1.));
#11480=DIRECTION('center_axis',(0.,0.,1.));
#11481=DIRECTION('ref_axis',(1.,0.,0.));
#11482=DIRECTION('',(0.,0.,1.));
#11483=DIRECTION('center_axis',(0.,0.,-1.));
#11484=DIRECTION('ref_axis',(1.,0.,0.));
#11485=DIRECTION('center_axis',(0.,0.,1.));
#11486=DIRECTION('ref_axis',(1.,0.,0.));
#11487=DIRECTION('',(0.,0.,1.));
#11488=DIRECTION('center_axis',(0.,0.,1.));
#11489=DIRECTION('ref_axis',(1.,0.,0.));
#11490=DIRECTION('',(1.,0.,0.));
#11491=DIRECTION('center_axis',(0.,0.,1.));
#11492=DIRECTION('ref_axis',(1.,0.,0.));
#11493=DIRECTION('center_axis',(0.,0.,1.));
#11494=DIRECTION('ref_axis',(1.,0.,0.));
#11495=DIRECTION('',(0.,0.,-1.));
#11496=DIRECTION('center_axis',(0.,0.,1.));
#11497=DIRECTION('ref_axis',(1.,0.,0.));
#11498=DIRECTION('',(0.,0.,1.));
#11499=DIRECTION('center_axis',(0.,0.,-1.));
#11500=DIRECTION('ref_axis',(1.,0.,0.));
#11501=DIRECTION('center_axis',(0.,0.,1.));
#11502=DIRECTION('ref_axis',(1.,0.,0.));
#11503=DIRECTION('',(0.,0.,1.));
#11504=DIRECTION('center_axis',(0.,-1.,0.));
#11505=DIRECTION('ref_axis',(0.,0.,-1.));
#11506=DIRECTION('',(-1.,0.,0.));
#11507=DIRECTION('',(-1.,0.,0.));
#11508=DIRECTION('',(0.,0.,1.));
#11509=DIRECTION('',(1.,0.,0.));
#11510=DIRECTION('',(0.,0.,-1.));
#11511=DIRECTION('',(-1.,0.,0.));
#11512=DIRECTION('center_axis',(0.,1.,0.));
#11513=DIRECTION('ref_axis',(0.,0.,1.));
#11514=DIRECTION('',(1.,0.,0.));
#11515=DIRECTION('',(1.,0.,0.));
#11516=DIRECTION('',(0.,0.,1.));
#11517=DIRECTION('',(1.,0.,0.));
#11518=DIRECTION('',(0.,0.,-1.));
#11519=DIRECTION('',(1.,0.,0.));
#11520=DIRECTION('center_axis',(-1.,0.,0.));
#11521=DIRECTION('ref_axis',(0.,0.,1.));
#11522=DIRECTION('',(0.,-1.,0.));
#11523=DIRECTION('',(0.,0.,1.));
#11524=DIRECTION('',(0.,1.,0.));
#11525=DIRECTION('',(0.,0.,-1.));
#11526=DIRECTION('',(0.,-1.,0.));
#11527=DIRECTION('',(0.,-1.,0.));
#11528=DIRECTION('',(0.,0.,1.));
#11529=DIRECTION('',(0.,-1.,0.));
#11530=DIRECTION('',(0.,0.,-1.));
#11531=DIRECTION('',(0.,-1.,0.));
#11532=DIRECTION('center_axis',(0.,0.,-1.));
#11533=DIRECTION('ref_axis',(0.,1.,0.));
#11534=DIRECTION('',(0.,1.,0.));
#11535=DIRECTION('',(1.,0.,0.));
#11536=DIRECTION('center_axis',(0.,-1.,0.));
#11537=DIRECTION('ref_axis',(0.,0.,-1.));
#11538=DIRECTION('',(0.,0.,-1.));
#11539=DIRECTION('',(1.,0.,0.));
#11540=DIRECTION('center_axis',(0.,0.,1.));
#11541=DIRECTION('ref_axis',(0.,-1.,0.));
#11542=DIRECTION('',(0.,-1.,0.));
#11543=DIRECTION('',(1.,0.,0.));
#11544=DIRECTION('center_axis',(0.,1.,0.));
#11545=DIRECTION('ref_axis',(0.,0.,1.));
#11546=DIRECTION('',(0.,0.,1.));
#11547=DIRECTION('',(1.,0.,0.));
#11548=DIRECTION('center_axis',(0.,0.,-1.));
#11549=DIRECTION('ref_axis',(0.,1.,0.));
#11550=DIRECTION('',(0.,1.,0.));
#11551=DIRECTION('center_axis',(0.,0.,-1.));
#11552=DIRECTION('ref_axis',(0.,1.,0.));
#11553=DIRECTION('',(0.,1.,0.));
#11554=DIRECTION('',(1.,0.,0.));
#11555=DIRECTION('center_axis',(0.,-1.,0.));
#11556=DIRECTION('ref_axis',(0.,0.,-1.));
#11557=DIRECTION('',(0.,0.,-1.));
#11558=DIRECTION('',(1.,0.,0.));
#11559=DIRECTION('center_axis',(0.,0.,-1.));
#11560=DIRECTION('ref_axis',(0.,1.,0.));
#11561=DIRECTION('',(0.,1.,0.));
#11562=DIRECTION('',(1.,0.,0.));
#11563=DIRECTION('center_axis',(0.,1.,0.));
#11564=DIRECTION('ref_axis',(0.,0.,1.));
#11565=DIRECTION('',(0.,0.,1.));
#11566=DIRECTION('',(1.,0.,0.));
#11567=DIRECTION('center_axis',(0.,0.,-1.));
#11568=DIRECTION('ref_axis',(0.,1.,0.));
#11569=DIRECTION('',(0.,1.,0.));
#11570=DIRECTION('center_axis',(1.,0.,0.));
#11571=DIRECTION('ref_axis',(0.,0.,-1.));
#14324=CARTESIAN_POINT('',(0.,0.,0.));
#14325=CARTESIAN_POINT('Origin',(1.5,-1.9,1.7));
#14326=CARTESIAN_POINT('',(1.56403124237433,-1.7,1.7));
#14327=CARTESIAN_POINT('',(1.43596875762567,-1.7,1.7));
#14328=CARTESIAN_POINT('',(0.75,-1.7,1.7));
#14329=CARTESIAN_POINT('Origin',(1.5,-1.9,1.7));
#14330=CARTESIAN_POINT('Origin',(1.5,-1.9,1.7));
#14331=CARTESIAN_POINT('',(1.56403124237433,-1.7,1.75));
#14332=CARTESIAN_POINT('',(1.56403124237433,-1.7,1.7));
#14333=CARTESIAN_POINT('',(1.29,-1.9,1.75));
#14334=CARTESIAN_POINT('Origin',(1.5,-1.9,1.75));
#14335=CARTESIAN_POINT('',(1.29,-1.9,2.4));
#14336=CARTESIAN_POINT('',(1.29,-1.9,1.7));
#14337=CARTESIAN_POINT('Origin',(1.5,-1.9,2.4));
#14338=CARTESIAN_POINT('',(1.43596875762567,-1.7,1.75));
#14339=CARTESIAN_POINT('Origin',(1.5,-1.9,1.75));
#14340=CARTESIAN_POINT('',(1.43596875762567,-1.7,1.7));
#14341=CARTESIAN_POINT('Origin',(-1.5,1.9,1.7));
#14342=CARTESIAN_POINT('',(-1.56403124237433,1.7,1.7));
#14343=CARTESIAN_POINT('',(-1.43596875762567,1.7,1.7));
#14344=CARTESIAN_POINT('',(-0.75,1.7,1.7));
#14345=CARTESIAN_POINT('Origin',(-1.5,1.9,1.7));
#14346=CARTESIAN_POINT('Origin',(-1.5,1.9,1.7));
#14347=CARTESIAN_POINT('',(-1.56403124237433,1.7,1.75));
#14348=CARTESIAN_POINT('',(-1.56403124237433,1.7,1.7));
#14349=CARTESIAN_POINT('',(-1.71,1.9,1.75));
#14350=CARTESIAN_POINT('Origin',(-1.5,1.9,1.75));
#14351=CARTESIAN_POINT('',(-1.71,1.9,2.4));
#14352=CARTESIAN_POINT('',(-1.71,1.9,1.7));
#14353=CARTESIAN_POINT('Origin',(-1.5,1.9,2.4));
#14354=CARTESIAN_POINT('',(-1.43596875762567,1.7,1.75));
#14355=CARTESIAN_POINT('Origin',(-1.5,1.9,1.75));
#14356=CARTESIAN_POINT('',(-1.43596875762567,1.7,1.7));
#14357=CARTESIAN_POINT('Origin',(-1.5,-1.9,1.7));
#14358=CARTESIAN_POINT('',(-1.43596875762567,-1.7,1.7));
#14359=CARTESIAN_POINT('',(-1.56403124237433,-1.7,1.7));
#14360=CARTESIAN_POINT('',(-0.75,-1.7,1.7));
#14361=CARTESIAN_POINT('Origin',(-1.5,-1.9,1.7));
#14362=CARTESIAN_POINT('Origin',(-1.5,-1.9,1.7));
#14363=CARTESIAN_POINT('',(-1.43596875762567,-1.7,1.75));
#14364=CARTESIAN_POINT('',(-1.43596875762567,-1.7,1.7));
#14365=CARTESIAN_POINT('',(-1.71,-1.9,1.75));
#14366=CARTESIAN_POINT('Origin',(-1.5,-1.9,1.75));
#14367=CARTESIAN_POINT('',(-1.71,-1.9,2.4));
#14368=CARTESIAN_POINT('',(-1.71,-1.9,1.7));
#14369=CARTESIAN_POINT('Origin',(-1.5,-1.9,2.4));
#14370=CARTESIAN_POINT('',(-1.56403124237433,-1.7,1.75));
#14371=CARTESIAN_POINT('Origin',(-1.5,-1.9,1.75));
#14372=CARTESIAN_POINT('',(-1.56403124237433,-1.7,1.7));
#14373=CARTESIAN_POINT('Origin',(1.5,1.9,1.7));
#14374=CARTESIAN_POINT('',(1.43596875762567,1.7,1.7));
#14375=CARTESIAN_POINT('',(1.56403124237433,1.7,1.7));
#14376=CARTESIAN_POINT('',(0.75,1.7,1.7));
#14377=CARTESIAN_POINT('Origin',(1.5,1.9,1.7));
#14378=CARTESIAN_POINT('Origin',(1.5,1.9,1.7));
#14379=CARTESIAN_POINT('',(1.43596875762567,1.7,1.75));
#14380=CARTESIAN_POINT('',(1.43596875762567,1.7,1.7));
#14381=CARTESIAN_POINT('',(1.29,1.9,1.75));
#14382=CARTESIAN_POINT('Origin',(1.5,1.9,1.75));
#14383=CARTESIAN_POINT('',(1.29,1.9,2.4));
#14384=CARTESIAN_POINT('',(1.29,1.9,1.7));
#14385=CARTESIAN_POINT('Origin',(1.5,1.9,2.4));
#14386=CARTESIAN_POINT('',(1.56403124237433,1.7,1.75));
#14387=CARTESIAN_POINT('Origin',(1.5,1.9,1.75));
#14388=CARTESIAN_POINT('',(1.56403124237433,1.7,1.7));
#14389=CARTESIAN_POINT('Origin',(0.,-1.7,1.75));
#14390=CARTESIAN_POINT('',(0.,-1.7,1.75));
#14391=CARTESIAN_POINT('',(-1.97,-1.7,1.75));
#14392=CARTESIAN_POINT('',(0.,-1.7,1.75));
#14393=CARTESIAN_POINT('',(-1.97,-1.7,0.43));
#14394=CARTESIAN_POINT('',(-1.97,-1.7,1.75));
#14395=CARTESIAN_POINT('',(1.97,-1.7,0.43));
#14396=CARTESIAN_POINT('',(0.,-1.7,0.43));
#14397=CARTESIAN_POINT('',(1.97,-1.7,1.75));
#14398=CARTESIAN_POINT('',(1.97,-1.7,1.75));
#14399=CARTESIAN_POINT('',(0.,-1.7,1.75));
#14400=CARTESIAN_POINT('Origin',(0.,1.7,0.43));
#14401=CARTESIAN_POINT('',(0.,1.7,1.75));
#14402=CARTESIAN_POINT('',(1.97,1.7,1.75));
#14403=CARTESIAN_POINT('',(0.,1.7,1.75));
#14404=CARTESIAN_POINT('',(1.97,1.7,0.43));
#14405=CARTESIAN_POINT('',(1.97,1.7,0.43));
#14406=CARTESIAN_POINT('',(-1.97,1.7,0.43));
#14407=CARTESIAN_POINT('',(0.,1.7,0.43));
#14408=CARTESIAN_POINT('',(-1.97,1.7,1.75));
#14409=CARTESIAN_POINT('',(-1.97,1.7,0.43));
#14410=CARTESIAN_POINT('',(0.,1.7,1.75));
#14411=CARTESIAN_POINT('Origin',(-1.97,0.,1.415));
#14412=CARTESIAN_POINT('',(-1.97,-2.35,1.75));
#14413=CARTESIAN_POINT('',(-1.97,-2.35,1.75));
#14414=CARTESIAN_POINT('',(-1.97,-2.35,2.4));
#14415=CARTESIAN_POINT('',(-1.97,-2.35,2.4));
#14416=CARTESIAN_POINT('',(-1.97,2.35,2.4));
#14417=CARTESIAN_POINT('',(-1.97,2.35,2.4));
#14418=CARTESIAN_POINT('',(-1.97,2.35,1.75));
#14419=CARTESIAN_POINT('',(-1.97,2.35,1.75));
#14420=CARTESIAN_POINT('',(-1.97,1.7,1.75));
#14421=CARTESIAN_POINT('',(-1.97,0.78,0.43));
#14422=CARTESIAN_POINT('',(-1.97,0.78,0.43));
#14423=CARTESIAN_POINT('',(-1.97,0.78,1.55));
#14424=CARTESIAN_POINT('',(-1.97,0.78,1.55));
#14425=CARTESIAN_POINT('',(-1.97,-0.78,1.55));
#14426=CARTESIAN_POINT('',(-1.97,-0.78,1.55));
#14427=CARTESIAN_POINT('',(-1.97,-0.78,0.43));
#14428=CARTESIAN_POINT('',(-1.97,-0.78,0.43));
#14429=CARTESIAN_POINT('',(-1.97,-1.7,0.43));
#14430=CARTESIAN_POINT('Origin',(0.,-2.35,1.75));
#14431=CARTESIAN_POINT('',(1.97,-2.35,1.75));
#14432=CARTESIAN_POINT('',(1.97,-2.35,1.75));
#14433=CARTESIAN_POINT('',(0.,-2.35,1.75));
#14434=CARTESIAN_POINT('Origin',(0.,-2.35,2.4));
#14435=CARTESIAN_POINT('',(1.97,-2.35,2.4));
#14436=CARTESIAN_POINT('',(1.97,-2.35,2.4));
#14437=CARTESIAN_POINT('',(0.,-2.35,2.4));
#14438=CARTESIAN_POINT('Origin',(0.,2.35,2.4));
#14439=CARTESIAN_POINT('',(1.97,2.35,2.4));
#14440=CARTESIAN_POINT('',(1.97,2.35,2.4));
#14441=CARTESIAN_POINT('',(0.,2.35,2.4));
#14442=CARTESIAN_POINT('Origin',(0.,2.35,1.75));
#14443=CARTESIAN_POINT('',(1.97,2.35,1.75));
#14444=CARTESIAN_POINT('',(1.97,2.35,1.75));
#14445=CARTESIAN_POINT('',(0.,2.35,1.75));
#14446=CARTESIAN_POINT('Origin',(0.,1.7,1.75));
#14447=CARTESIAN_POINT('',(1.97,1.7,1.75));
#14448=CARTESIAN_POINT('Origin',(0.,0.78,0.43));
#14449=CARTESIAN_POINT('',(1.97,0.78,0.43));
#14450=CARTESIAN_POINT('',(1.97,0.78,0.43));
#14451=CARTESIAN_POINT('',(0.,0.78,0.43));
#14452=CARTESIAN_POINT('Origin',(0.,0.78,1.55));
#14453=CARTESIAN_POINT('',(1.97,0.78,1.55));
#14454=CARTESIAN_POINT('',(1.97,0.78,1.55));
#14455=CARTESIAN_POINT('',(0.,0.78,1.55));
#14456=CARTESIAN_POINT('Origin',(0.,-0.78,1.55));
#14457=CARTESIAN_POINT('',(1.97,-0.78,1.55));
#14458=CARTESIAN_POINT('',(1.97,-0.78,1.55));
#14459=CARTESIAN_POINT('',(0.,-0.78,1.55));
#14460=CARTESIAN_POINT('Origin',(0.,-0.78,0.43));
#14461=CARTESIAN_POINT('',(1.97,-0.78,0.43));
#14462=CARTESIAN_POINT('',(1.97,-0.78,0.43));
#14463=CARTESIAN_POINT('',(0.,-0.78,0.43));
#14464=CARTESIAN_POINT('Origin',(0.,-1.7,0.43));
#14465=CARTESIAN_POINT('',(1.97,-1.7,0.43));
#14466=CARTESIAN_POINT('Origin',(1.97,0.,1.415));
#14819=UNCERTAINTY_MEASURE_WITH_UNIT(LENGTH_MEASURE(0.001),#14879,
'DISTANCE_ACCURACY_VALUE',
'Maximum model space distance between geometric entities at asserted c
onnectivities');
#14824=UNCERTAINTY_MEASURE_WITH_UNIT(LENGTH_MEASURE(0.001),#14879,
'DISTANCE_ACCURACY_VALUE',
'Maximum model space distance between geometric entities at asserted c
onnectivities');
#14873=(
GEOMETRIC_REPRESENTATION_CONTEXT(3)
GLOBAL_UNCERTAINTY_ASSIGNED_CONTEXT((#14819))
GLOBAL_UNIT_ASSIGNED_CONTEXT((#14879,#14881,#14882))
REPRESENTATION_CONTEXT('','3D')
);
#14878=(
GEOMETRIC_REPRESENTATION_CONTEXT(3)
GLOBAL_UNCERTAINTY_ASSIGNED_CONTEXT((#14824))
GLOBAL_UNIT_ASSIGNED_CONTEXT((#14879,#14881,#14882))
REPRESENTATION_CONTEXT('','3D')
);
#14879=(
LENGTH_UNIT()
NAMED_UNIT(*)
SI_UNIT(.CENTI.,.METRE.)
);
#14881=(
NAMED_UNIT(*)
PLANE_ANGLE_UNIT()
SI_UNIT($,.RADIAN.)
);
#14882=(
NAMED_UNIT(*)
SI_UNIT($,.STERADIAN.)
SOLID_ANGLE_UNIT()
);
#14931=SHAPE_DEFINITION_REPRESENTATION(#14993,#15116);
#14993=PRODUCT_DEFINITION_SHAPE('',$,#15170);
#15116=SHAPE_REPRESENTATION('',(#9218),#14873);
#15121=PRODUCT_DEFINITION_CONTEXT('part definition',#15282,'design');
#15170=PRODUCT_DEFINITION('Block','Block',#15223,#15121);
#15223=PRODUCT_DEFINITION_FORMATION('',$,#15332);
#15282=APPLICATION_CONTEXT(
'Core Data for Automotive Mechanical Design Process');
#15283=PRODUCT_CONTEXT('part definition',#15282,'mechanical');
#15332=PRODUCT('Block','Block','Block',(#15283));
#15379=COLOUR_RGB('Dark Blue',0.08,0.2,0.34);
#15380=FILL_AREA_STYLE_COLOUR('',#15379);
#15381=FILL_AREA_STYLE('',(#15380));
#15382=SURFACE_STYLE_FILL_AREA(#15381);
#15383=SURFACE_SIDE_STYLE('',(#15382));
#15384=SURFACE_STYLE_USAGE(.BOTH.,#15383);
#15385=PRESENTATION_STYLE_ASSIGNMENT((#15384));
ENDSEC;
END-ISO-10303-21;
